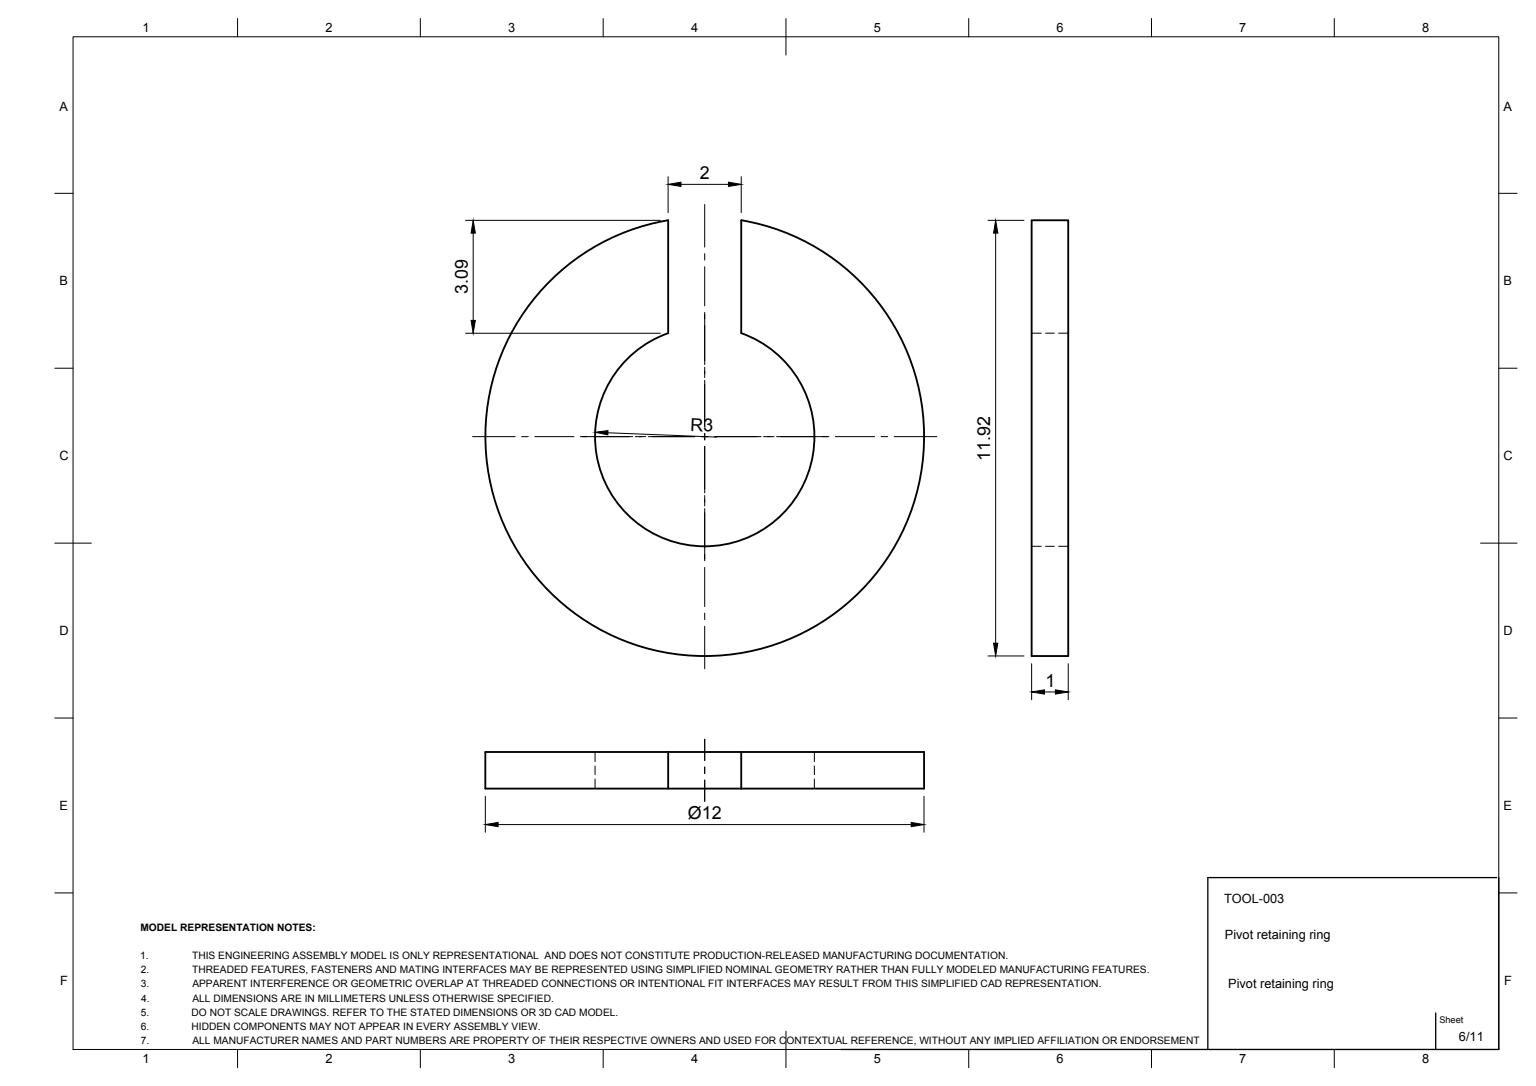
ISO-10303-21;
HEADER;
/* Generated by software containing ST-Developer
 * from STEP Tools, Inc. (www.steptools.com) 
 */

FILE_DESCRIPTION(
/* description */ (''),
/* implementation_level */ '2;1');

FILE_NAME(
/* name */ 'Pivot retaining ring.step',
/* time_stamp */ '2026-11-10T05:20:16-08:00',
/* author */ (''),
/* organization */ (''),
/* preprocessor_version */ 'ST-DEVELOPER v20.2',
/* originating_system */ 'Autodesk Translation Framework v15.17.0.0',
/* authorisation */ '');

FILE_SCHEMA (('AUTOMOTIVE_DESIGN { 1 0 10303 214 3 1 1 }'));
ENDSEC;

DATA;
#10=MECHANICAL_DESIGN_GEOMETRIC_PRESENTATION_REPRESENTATION('',(#115),#24809);
#95=SHAPE_REPRESENTATION_RELATIONSHIP('SRR','None',#24858,#105);
#105=ADVANCED_BREP_SHAPE_REPRESENTATION('',(#125),#24801);
#115=STYLED_ITEM('',(#24921),#125);
#125=MANIFOLD_SOLID_BREP('Body1',#9892);
#1192=PLANE('',#10250);
#1193=PLANE('',#10251);
#1194=PLANE('',#10252);
#1195=PLANE('',#10259);
#1523=FACE_OUTER_BOUND('',#2091,.T.);
#1524=FACE_OUTER_BOUND('',#2092,.T.);
#1525=FACE_OUTER_BOUND('',#2093,.T.);
#1526=FACE_OUTER_BOUND('',#2094,.T.);
#1527=FACE_OUTER_BOUND('',#2095,.T.);
#1528=FACE_OUTER_BOUND('',#2096,.T.);
#2091=EDGE_LOOP('',(#7473,#7474,#7475,#7476));
#2092=EDGE_LOOP('',(#7477,#7478,#7479,#7480));
#2093=EDGE_LOOP('',(#7481,#7482,#7483,#7484));
#2094=EDGE_LOOP('',(#7485,#7486,#7487,#7488));
#2095=EDGE_LOOP('',(#7489,#7490,#7491,#7492));
#2096=EDGE_LOOP('',(#7493,#7494,#7495,#7496));
#2731=LINE('',#14914,#3319);
#2732=LINE('',#14916,#3320);
#2733=LINE('',#14918,#3321);
#2734=LINE('',#14919,#3322);
#2735=LINE('',#14923,#3323);
#2736=LINE('',#14925,#3324);
#2737=LINE('',#14927,#3325);
#2738=LINE('',#14928,#3326);
#3319=VECTOR('',#11403,1.);
#3320=VECTOR('',#11404,1.);
#3321=VECTOR('',#11405,1.);
#3322=VECTOR('',#11406,1.);
#3323=VECTOR('',#11409,1.);
#3324=VECTOR('',#11410,1.);
#3325=VECTOR('',#11411,1.);
#3326=VECTOR('',#11412,1.);
#3687=CIRCLE('',#10253,0.6);
#3688=CIRCLE('',#10254,0.3);
#3689=CIRCLE('',#10256,0.3);
#3690=CIRCLE('',#10258,0.6);
#4231=VERTEX_POINT('',#14912);
#4232=VERTEX_POINT('',#14913);
#4233=VERTEX_POINT('',#14915);
#4234=VERTEX_POINT('',#14917);
#4235=VERTEX_POINT('',#14921);
#4236=VERTEX_POINT('',#14922);
#4237=VERTEX_POINT('',#14924);
#4238=VERTEX_POINT('',#14926);
#5395=EDGE_CURVE('',#4231,#4232,#2731,.T.);
#5396=EDGE_CURVE('',#4233,#4231,#2732,.T.);
#5397=EDGE_CURVE('',#4234,#4233,#2733,.T.);
#5398=EDGE_CURVE('',#4232,#4234,#2734,.T.);
#5399=EDGE_CURVE('',#4235,#4236,#2735,.T.);
#5400=EDGE_CURVE('',#4237,#4235,#2736,.T.);
#5401=EDGE_CURVE('',#4238,#4237,#2737,.T.);
#5402=EDGE_CURVE('',#4236,#4238,#2738,.T.);
#5403=EDGE_CURVE('',#4233,#4238,#3687,.T.);
#5404=EDGE_CURVE('',#4236,#4231,#3688,.T.);
#5405=EDGE_CURVE('',#4235,#4232,#3689,.T.);
#5406=EDGE_CURVE('',#4234,#4237,#3690,.T.);
#7473=ORIENTED_EDGE('',*,*,#5395,.F.);
#7474=ORIENTED_EDGE('',*,*,#5396,.F.);
#7475=ORIENTED_EDGE('',*,*,#5397,.F.);
#7476=ORIENTED_EDGE('',*,*,#5398,.F.);
#7477=ORIENTED_EDGE('',*,*,#5399,.F.);
#7478=ORIENTED_EDGE('',*,*,#5400,.F.);
#7479=ORIENTED_EDGE('',*,*,#5401,.F.);
#7480=ORIENTED_EDGE('',*,*,#5402,.F.);
#7481=ORIENTED_EDGE('',*,*,#5402,.T.);
#7482=ORIENTED_EDGE('',*,*,#5403,.F.);
#7483=ORIENTED_EDGE('',*,*,#5396,.T.);
#7484=ORIENTED_EDGE('',*,*,#5404,.F.);
#7485=ORIENTED_EDGE('',*,*,#5399,.T.);
#7486=ORIENTED_EDGE('',*,*,#5404,.T.);
#7487=ORIENTED_EDGE('',*,*,#5395,.T.);
#7488=ORIENTED_EDGE('',*,*,#5405,.F.);
#7489=ORIENTED_EDGE('',*,*,#5401,.T.);
#7490=ORIENTED_EDGE('',*,*,#5406,.F.);
#7491=ORIENTED_EDGE('',*,*,#5397,.T.);
#7492=ORIENTED_EDGE('',*,*,#5403,.T.);
#7493=ORIENTED_EDGE('',*,*,#5400,.T.);
#7494=ORIENTED_EDGE('',*,*,#5405,.T.);
#7495=ORIENTED_EDGE('',*,*,#5398,.T.);
#7496=ORIENTED_EDGE('',*,*,#5406,.T.);
#9211=CYLINDRICAL_SURFACE('',#10255,0.3);
#9212=CYLINDRICAL_SURFACE('',#10257,0.6);
#9549=ADVANCED_FACE('',(#1523),#1192,.F.);
#9550=ADVANCED_FACE('',(#1524),#1193,.F.);
#9551=ADVANCED_FACE('',(#1525),#1194,.F.);
#9552=ADVANCED_FACE('',(#1526),#9211,.F.);
#9553=ADVANCED_FACE('',(#1527),#9212,.T.);
#9554=ADVANCED_FACE('',(#1528),#1195,.T.);
#9892=CLOSED_SHELL('',(#9549,#9550,#9551,#9552,#9553,#9554));
#10249=AXIS2_PLACEMENT_3D('',#14910,#11399,#11400);
#10250=AXIS2_PLACEMENT_3D('',#14911,#11401,#11402);
#10251=AXIS2_PLACEMENT_3D('',#14920,#11407,#11408);
#10252=AXIS2_PLACEMENT_3D('',#14929,#11413,#11414);
#10253=AXIS2_PLACEMENT_3D('',#14930,#11415,#11416);
#10254=AXIS2_PLACEMENT_3D('',#14931,#11417,#11418);
#10255=AXIS2_PLACEMENT_3D('',#14932,#11419,#11420);
#10256=AXIS2_PLACEMENT_3D('',#14933,#11421,#11422);
#10257=AXIS2_PLACEMENT_3D('',#14934,#11423,#11424);
#10258=AXIS2_PLACEMENT_3D('',#14935,#11425,#11426);
#10259=AXIS2_PLACEMENT_3D('',#14936,#11427,#11428);
#11399=DIRECTION('axis',(0.,0.,1.));
#11400=DIRECTION('refdir',(1.,0.,0.));
#11401=DIRECTION('center_axis',(-1.,0.,0.));
#11402=DIRECTION('ref_axis',(0.,1.,0.));
#11403=DIRECTION('',(0.,0.,1.));
#11404=DIRECTION('',(0.,-1.,0.));
#11405=DIRECTION('',(0.,0.,-1.));
#11406=DIRECTION('',(0.,1.,0.));
#11407=DIRECTION('center_axis',(1.,0.,0.));
#11408=DIRECTION('ref_axis',(0.,-1.,0.));
#11409=DIRECTION('',(0.,0.,-1.));
#11410=DIRECTION('',(0.,-1.,0.));
#11411=DIRECTION('',(0.,0.,1.));
#11412=DIRECTION('',(0.,1.,0.));
#11413=DIRECTION('center_axis',(0.,0.,1.));
#11414=DIRECTION('ref_axis',(1.,0.,0.));
#11415=DIRECTION('center_axis',(0.,0.,1.));
#11416=DIRECTION('ref_axis',(1.,0.,0.));
#11417=DIRECTION('center_axis',(0.,0.,-1.));
#11418=DIRECTION('ref_axis',(1.,0.,0.));
#11419=DIRECTION('center_axis',(0.,0.,1.));
#11420=DIRECTION('ref_axis',(6.12323399573677E-17,-1.,0.));
#11421=DIRECTION('center_axis',(0.,0.,-1.));
#11422=DIRECTION('ref_axis',(1.,0.,0.));
#11423=DIRECTION('center_axis',(0.,0.,1.));
#11424=DIRECTION('ref_axis',(6.12323399573677E-17,-1.,0.));
#11425=DIRECTION('center_axis',(0.,0.,1.));
#11426=DIRECTION('ref_axis',(1.,0.,0.));
#11427=DIRECTION('center_axis',(0.,0.,1.));
#11428=DIRECTION('ref_axis',(1.,0.,0.));
#14910=CARTESIAN_POINT('',(0.,0.,0.));
#14911=CARTESIAN_POINT('Origin',(-0.1,0.,0.1));
#14912=CARTESIAN_POINT('',(-0.1,0.282842712474619,0.));
#14913=CARTESIAN_POINT('',(-0.1,0.282842712474619,0.1));
#14914=CARTESIAN_POINT('',(-0.1,0.282842712474619,0.));
#14915=CARTESIAN_POINT('',(-0.1,0.591607978309962,0.));
#14916=CARTESIAN_POINT('',(-0.1,0.,0.));
#14917=CARTESIAN_POINT('',(-0.1,0.591607978309962,0.1));
#14918=CARTESIAN_POINT('',(-0.1,0.591607978309962,0.));
#14919=CARTESIAN_POINT('',(-0.1,0.,0.1));
#14920=CARTESIAN_POINT('Origin',(0.1,1.2,0.1));
#14921=CARTESIAN_POINT('',(0.1,0.282842712474619,0.1));
#14922=CARTESIAN_POINT('',(0.1,0.282842712474619,0.));
#14923=CARTESIAN_POINT('',(0.1,0.282842712474619,0.));
#14924=CARTESIAN_POINT('',(0.1,0.591607978309962,0.1));
#14925=CARTESIAN_POINT('',(0.1,0.6,0.1));
#14926=CARTESIAN_POINT('',(0.1,0.591607978309962,0.));
#14927=CARTESIAN_POINT('',(0.1,0.591607978309962,0.));
#14928=CARTESIAN_POINT('',(0.1,0.6,0.));
#14929=CARTESIAN_POINT('Origin',(0.,0.,0.));
#14930=CARTESIAN_POINT('Origin',(0.,0.,0.));
#14931=CARTESIAN_POINT('Origin',(0.,0.,0.));
#14932=CARTESIAN_POINT('Origin',(0.,0.,0.));
#14933=CARTESIAN_POINT('Origin',(0.,0.,0.1));
#14934=CARTESIAN_POINT('Origin',(0.,0.,0.));
#14935=CARTESIAN_POINT('Origin',(0.,0.,0.1));
#14936=CARTESIAN_POINT('Origin',(0.,0.,0.1));
#24788=UNCERTAINTY_MEASURE_WITH_UNIT(LENGTH_MEASURE(0.001),#24810,
'DISTANCE_ACCURACY_VALUE',
'Maximum model space distance between geometric entities at asserted c
onnectivities');
#24796=UNCERTAINTY_MEASURE_WITH_UNIT(LENGTH_MEASURE(0.001),#24810,
'DISTANCE_ACCURACY_VALUE',
'Maximum model space distance between geometric entities at asserted c
onnectivities');
#24801=(
GEOMETRIC_REPRESENTATION_CONTEXT(3)
GLOBAL_UNCERTAINTY_ASSIGNED_CONTEXT((#24788))
GLOBAL_UNIT_ASSIGNED_CONTEXT((#24810,#24812,#24813))
REPRESENTATION_CONTEXT('','3D')
);
#24809=(
GEOMETRIC_REPRESENTATION_CONTEXT(3)
GLOBAL_UNCERTAINTY_ASSIGNED_CONTEXT((#24796))
GLOBAL_UNIT_ASSIGNED_CONTEXT((#24810,#24812,#24813))
REPRESENTATION_CONTEXT('','3D')
);
#24810=(
LENGTH_UNIT()
NAMED_UNIT(*)
SI_UNIT(.CENTI.,.METRE.)
);
#24812=(
NAMED_UNIT(*)
PLANE_ANGLE_UNIT()
SI_UNIT($,.RADIAN.)
);
#24813=(
NAMED_UNIT(*)
SI_UNIT($,.STERADIAN.)
SOLID_ANGLE_UNIT()
);
#24818=SHAPE_DEFINITION_REPRESENTATION(#24830,#24858);
#24830=PRODUCT_DEFINITION_SHAPE('',$,#24871);
#24858=SHAPE_REPRESENTATION('',(#10249),#24801);
#24866=PRODUCT_DEFINITION_CONTEXT('part definition',#24904,'design');
#24871=PRODUCT_DEFINITION('Pivot retaining ring','Pivot retaining ring',
#24883,#24866);
#24883=PRODUCT_DEFINITION_FORMATION('',$,#24910);
#24904=APPLICATION_CONTEXT(
'Core Data for Automotive Mechanical Design Process');
#24905=PRODUCT_CONTEXT('part definition',#24904,'mechanical');
#24910=PRODUCT('Pivot retaining ring','Pivot retaining ring',$,(#24905));
#24921=PRESENTATION_STYLE_ASSIGNMENT((#24929));
#24929=SURFACE_STYLE_USAGE(.BOTH.,#24937);
#24937=SURFACE_SIDE_STYLE('',(#24945));
#24945=SURFACE_STYLE_FILL_AREA(#24953);
#24953=FILL_AREA_STYLE('Dark gray',(#24961));
#24961=FILL_AREA_STYLE_COLOUR('Dark gray',#24969);
#24969=COLOUR_RGB('Dark gray',0.250980392156863,0.282352941176471,0.32156862745098);
ENDSEC;
END-ISO-10303-21;
